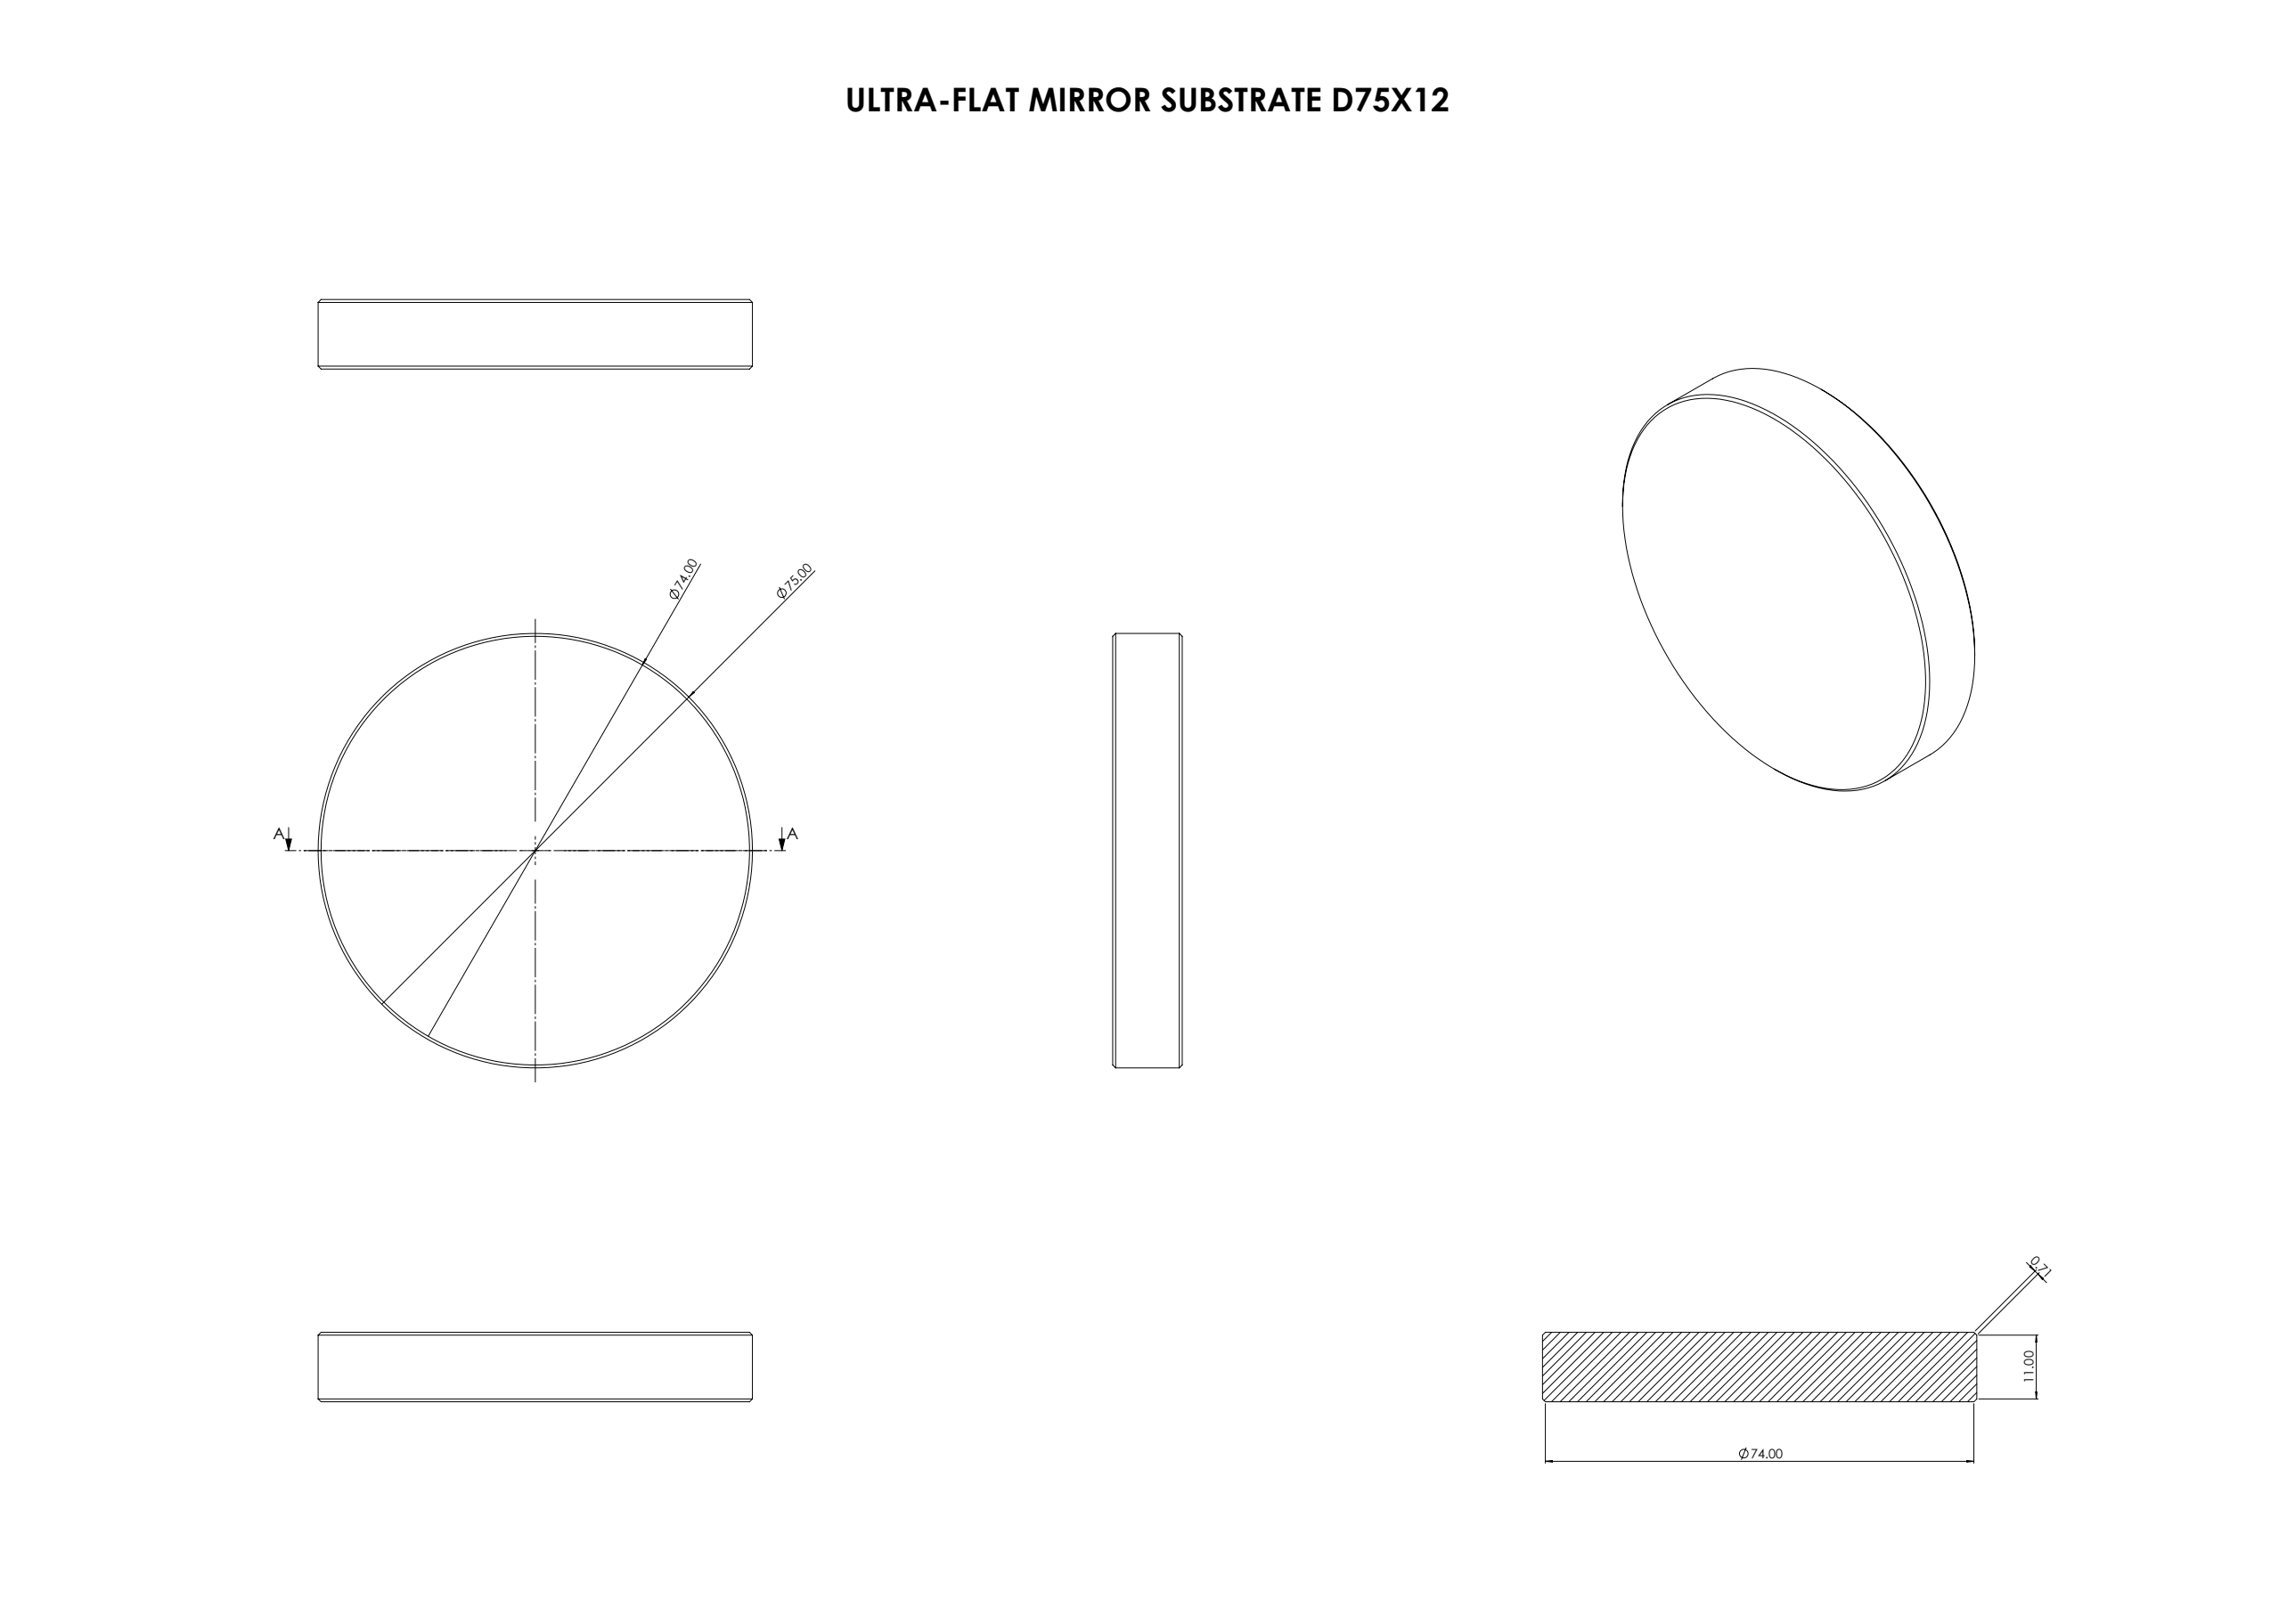
ISO-10303-21;
HEADER;
/* Generated by software containing ST-Developer
 * from STEP Tools, Inc. (www.steptools.com) 
 */

FILE_DESCRIPTION(
/* description */ (''),
/* implementation_level */ '2;1');

FILE_NAME(
/* name */ '05_Ultra-Flat_Mirror_Substrate_D75x12.step',
/* time_stamp */ '2026-10-19T22:59:19-07:00',
/* author */ (''),
/* organization */ (''),
/* preprocessor_version */ 'ST-DEVELOPER v20.2',
/* originating_system */ 'Autodesk Translation Framework v15.15.0.0',
/* authorisation */ '');

FILE_SCHEMA (('AUTOMOTIVE_DESIGN { 1 0 10303 214 3 1 1 }'));
ENDSEC;

DATA;
#10=MECHANICAL_DESIGN_GEOMETRIC_PRESENTATION_REPRESENTATION('',(#917),#53650);
#885=SHAPE_REPRESENTATION_RELATIONSHIP('SRR','None',#53730,#901);
#901=ADVANCED_BREP_SHAPE_REPRESENTATION('',(#933),#53640);
#917=STYLED_ITEM('',(#53944),#933);
#933=MANIFOLD_SOLID_BREP('Mirror Substrate',#23309);
#1031=CYLINDRICAL_SURFACE('',#24336,3.75);
#1668=PLANE('',#24339);
#1669=PLANE('',#24342);
#2706=FACE_OUTER_BOUND('',#4139,.T.);
#2707=FACE_OUTER_BOUND('',#4140,.T.);
#2708=FACE_OUTER_BOUND('',#4141,.T.);
#2709=FACE_OUTER_BOUND('',#4142,.T.);
#2710=FACE_OUTER_BOUND('',#4143,.T.);
#4139=EDGE_LOOP('',(#17161,#17162,#17163,#17164,#17165));
#4140=EDGE_LOOP('',(#17166,#17167,#17168,#17169,#17170,#17171));
#4141=EDGE_LOOP('',(#17172));
#4142=EDGE_LOOP('',(#17173,#17174,#17175,#17176,#17177));
#4143=EDGE_LOOP('',(#17178));
#5423=CIRCLE('',#24333,3.7);
#5424=CIRCLE('',#24334,3.75);
#5425=CIRCLE('',#24335,3.75);
#5426=CIRCLE('',#24337,3.75);
#5427=CIRCLE('',#24338,3.75);
#5428=CIRCLE('',#24341,3.7);
#6488=LINE('',#35483,#8333);
#6489=LINE('',#35489,#8334);
#6490=LINE('',#35496,#8335);
#8333=VECTOR('',#27966,3.725);
#8334=VECTOR('',#27973,3.75);
#8335=VECTOR('',#27982,3.725);
#10182=VERTEX_POINT('',#35480);
#10183=VERTEX_POINT('',#35482);
#10184=VERTEX_POINT('',#35484);
#10185=VERTEX_POINT('',#35488);
#10186=VERTEX_POINT('',#35490);
#10187=VERTEX_POINT('',#35495);
#12758=EDGE_CURVE('',#10182,#10182,#5423,.T.);
#12759=EDGE_CURVE('',#10182,#10183,#6488,.T.);
#12760=EDGE_CURVE('',#10183,#10184,#5424,.T.);
#12761=EDGE_CURVE('',#10184,#10183,#5425,.T.);
#12762=EDGE_CURVE('',#10184,#10185,#6489,.T.);
#12763=EDGE_CURVE('',#10186,#10185,#5426,.T.);
#12764=EDGE_CURVE('',#10185,#10186,#5427,.T.);
#12765=EDGE_CURVE('',#10186,#10187,#6490,.T.);
#12766=EDGE_CURVE('',#10187,#10187,#5428,.T.);
#17161=ORIENTED_EDGE('',*,*,#12758,.T.);
#17162=ORIENTED_EDGE('',*,*,#12759,.T.);
#17163=ORIENTED_EDGE('',*,*,#12760,.T.);
#17164=ORIENTED_EDGE('',*,*,#12761,.T.);
#17165=ORIENTED_EDGE('',*,*,#12759,.F.);
#17166=ORIENTED_EDGE('',*,*,#12760,.F.);
#17167=ORIENTED_EDGE('',*,*,#12761,.F.);
#17168=ORIENTED_EDGE('',*,*,#12762,.T.);
#17169=ORIENTED_EDGE('',*,*,#12763,.F.);
#17170=ORIENTED_EDGE('',*,*,#12764,.F.);
#17171=ORIENTED_EDGE('',*,*,#12762,.F.);
#17172=ORIENTED_EDGE('',*,*,#12758,.F.);
#17173=ORIENTED_EDGE('',*,*,#12763,.T.);
#17174=ORIENTED_EDGE('',*,*,#12764,.T.);
#17175=ORIENTED_EDGE('',*,*,#12765,.T.);
#17176=ORIENTED_EDGE('',*,*,#12766,.T.);
#17177=ORIENTED_EDGE('',*,*,#12765,.F.);
#17178=ORIENTED_EDGE('',*,*,#12766,.F.);
#21939=CONICAL_SURFACE('',#24332,3.725,0.785398163397446);
#21940=CONICAL_SURFACE('',#24340,3.725,0.785398163397446);
#22445=ADVANCED_FACE('',(#2706),#21939,.T.);
#22446=ADVANCED_FACE('',(#2707),#1031,.T.);
#22447=ADVANCED_FACE('',(#2708),#1668,.T.);
#22448=ADVANCED_FACE('',(#2709),#21940,.T.);
#22449=ADVANCED_FACE('',(#2710),#1669,.T.);
#23309=CLOSED_SHELL('',(#22445,#22446,#22447,#22448,#22449));
#24331=AXIS2_PLACEMENT_3D('',#35478,#27960,#27961);
#24332=AXIS2_PLACEMENT_3D('',#35479,#27962,#27963);
#24333=AXIS2_PLACEMENT_3D('',#35481,#27964,#27965);
#24334=AXIS2_PLACEMENT_3D('',#35485,#27967,#27968);
#24335=AXIS2_PLACEMENT_3D('',#35486,#27969,#27970);
#24336=AXIS2_PLACEMENT_3D('',#35487,#27971,#27972);
#24337=AXIS2_PLACEMENT_3D('',#35491,#27974,#27975);
#24338=AXIS2_PLACEMENT_3D('',#35492,#27976,#27977);
#24339=AXIS2_PLACEMENT_3D('',#35493,#27978,#27979);
#24340=AXIS2_PLACEMENT_3D('',#35494,#27980,#27981);
#24341=AXIS2_PLACEMENT_3D('',#35497,#27983,#27984);
#24342=AXIS2_PLACEMENT_3D('',#35498,#27985,#27986);
#27960=DIRECTION('axis',(0.,0.,1.));
#27961=DIRECTION('refdir',(1.,0.,0.));
#27962=DIRECTION('center_axis',(0.,0.,-1.));
#27963=DIRECTION('ref_axis',(-1.,0.,0.));
#27964=DIRECTION('center_axis',(0.,0.,-1.));
#27965=DIRECTION('ref_axis',(-1.,0.,0.));
#27966=DIRECTION('',(0.707106781186546,8.65956056235491E-17,-0.707106781186549));
#27967=DIRECTION('center_axis',(0.,0.,1.));
#27968=DIRECTION('ref_axis',(-1.,0.,0.));
#27969=DIRECTION('center_axis',(0.,0.,1.));
#27970=DIRECTION('ref_axis',(-1.,0.,0.));
#27971=DIRECTION('center_axis',(0.,0.,1.));
#27972=DIRECTION('ref_axis',(1.,0.,0.));
#27973=DIRECTION('',(0.,0.,-1.));
#27974=DIRECTION('center_axis',(0.,0.,-1.));
#27975=DIRECTION('ref_axis',(-1.,0.,0.));
#27976=DIRECTION('center_axis',(0.,0.,-1.));
#27977=DIRECTION('ref_axis',(-1.,0.,0.));
#27978=DIRECTION('center_axis',(0.,0.,1.));
#27979=DIRECTION('ref_axis',(1.,0.,0.));
#27980=DIRECTION('center_axis',(0.,0.,1.));
#27981=DIRECTION('ref_axis',(-1.,0.,0.));
#27982=DIRECTION('',(-0.707106781186546,-8.65956056235491E-17,-0.707106781186549));
#27983=DIRECTION('center_axis',(0.,0.,1.));
#27984=DIRECTION('ref_axis',(-1.,0.,0.));
#27985=DIRECTION('center_axis',(0.,0.,-1.));
#27986=DIRECTION('ref_axis',(-1.,0.,0.));
#35478=CARTESIAN_POINT('',(0.,0.,0.));
#35479=CARTESIAN_POINT('Origin',(0.,0.,1.175));
#35480=CARTESIAN_POINT('',(3.7,-4.53119315684521E-16,1.2));
#35481=CARTESIAN_POINT('Origin',(0.,0.,1.2));
#35482=CARTESIAN_POINT('',(3.75,4.59242549680257E-16,1.15));
#35483=CARTESIAN_POINT('',(3.725,4.56180932682389E-16,1.175));
#35484=CARTESIAN_POINT('',(-3.75,-4.59242549680257E-16,1.15));
#35485=CARTESIAN_POINT('Origin',(0.,0.,1.15));
#35486=CARTESIAN_POINT('Origin',(0.,0.,1.15));
#35487=CARTESIAN_POINT('Origin',(0.,0.,0.6));
#35488=CARTESIAN_POINT('',(-3.75,-4.59242549680257E-16,0.05));
#35489=CARTESIAN_POINT('',(-3.75,-4.59242549680257E-16,0.6));
#35490=CARTESIAN_POINT('',(3.75,-4.59242549680257E-16,0.05));
#35491=CARTESIAN_POINT('Origin',(0.,0.,0.05));
#35492=CARTESIAN_POINT('Origin',(0.,0.,0.05));
#35493=CARTESIAN_POINT('Origin',(0.,0.,1.2));
#35494=CARTESIAN_POINT('Origin',(0.,0.,0.025));
#35495=CARTESIAN_POINT('',(3.7,4.53119315684521E-16,0.));
#35496=CARTESIAN_POINT('',(3.725,4.56180932682389E-16,0.025));
#35497=CARTESIAN_POINT('Origin',(0.,0.,0.));
#35498=CARTESIAN_POINT('Origin',(3.75,0.,0.));
#53622=UNCERTAINTY_MEASURE_WITH_UNIT(LENGTH_MEASURE(0.001),#53651,
'DISTANCE_ACCURACY_VALUE',
'Maximum model space distance between geometric entities at asserted c
onnectivities');
#53632=UNCERTAINTY_MEASURE_WITH_UNIT(LENGTH_MEASURE(0.001),#53651,
'DISTANCE_ACCURACY_VALUE',
'Maximum model space distance between geometric entities at asserted c
onnectivities');
#53640=(
GEOMETRIC_REPRESENTATION_CONTEXT(3)
GLOBAL_UNCERTAINTY_ASSIGNED_CONTEXT((#53622))
GLOBAL_UNIT_ASSIGNED_CONTEXT((#53651,#53653,#53654))
REPRESENTATION_CONTEXT('','3D')
);
#53650=(
GEOMETRIC_REPRESENTATION_CONTEXT(3)
GLOBAL_UNCERTAINTY_ASSIGNED_CONTEXT((#53632))
GLOBAL_UNIT_ASSIGNED_CONTEXT((#53651,#53653,#53654))
REPRESENTATION_CONTEXT('','3D')
);
#53651=(
LENGTH_UNIT()
NAMED_UNIT(*)
SI_UNIT(.CENTI.,.METRE.)
);
#53653=(
NAMED_UNIT(*)
PLANE_ANGLE_UNIT()
SI_UNIT($,.RADIAN.)
);
#53654=(
NAMED_UNIT(*)
SI_UNIT($,.STERADIAN.)
SOLID_ANGLE_UNIT()
);
#53662=SHAPE_DEFINITION_REPRESENTATION(#53679,#53730);
#53679=PRODUCT_DEFINITION_SHAPE('',$,#53748);
#53730=SHAPE_REPRESENTATION('',(#24331),#53640);
#53740=PRODUCT_DEFINITION_CONTEXT('part definition',#53793,'design');
#53748=PRODUCT_DEFINITION('2026-10-18-22-44-39-866',
'05_Ultra-Flat_Mirror_Substrate_D75x12',#53765,#53740);
#53765=PRODUCT_DEFINITION_FORMATION('',$,#53802);
#53793=APPLICATION_CONTEXT(
'Core Data for Automotive Mechanical Design Process');
#53794=PRODUCT_CONTEXT('part definition',#53793,'mechanical');
#53802=PRODUCT('2026-10-18-22-44-39-866',
'05_Ultra-Flat_Mirror_Substrate_D75x12',$,(#53794));
#53938=COLOUR_RGB('Light Blue',0.38,0.62,0.78);
#53939=FILL_AREA_STYLE_COLOUR('',#53938);
#53940=FILL_AREA_STYLE('',(#53939));
#53941=SURFACE_STYLE_FILL_AREA(#53940);
#53942=SURFACE_SIDE_STYLE('',(#53941));
#53943=SURFACE_STYLE_USAGE(.BOTH.,#53942);
#53944=PRESENTATION_STYLE_ASSIGNMENT((#53943));
ENDSEC;
END-ISO-10303-21;
